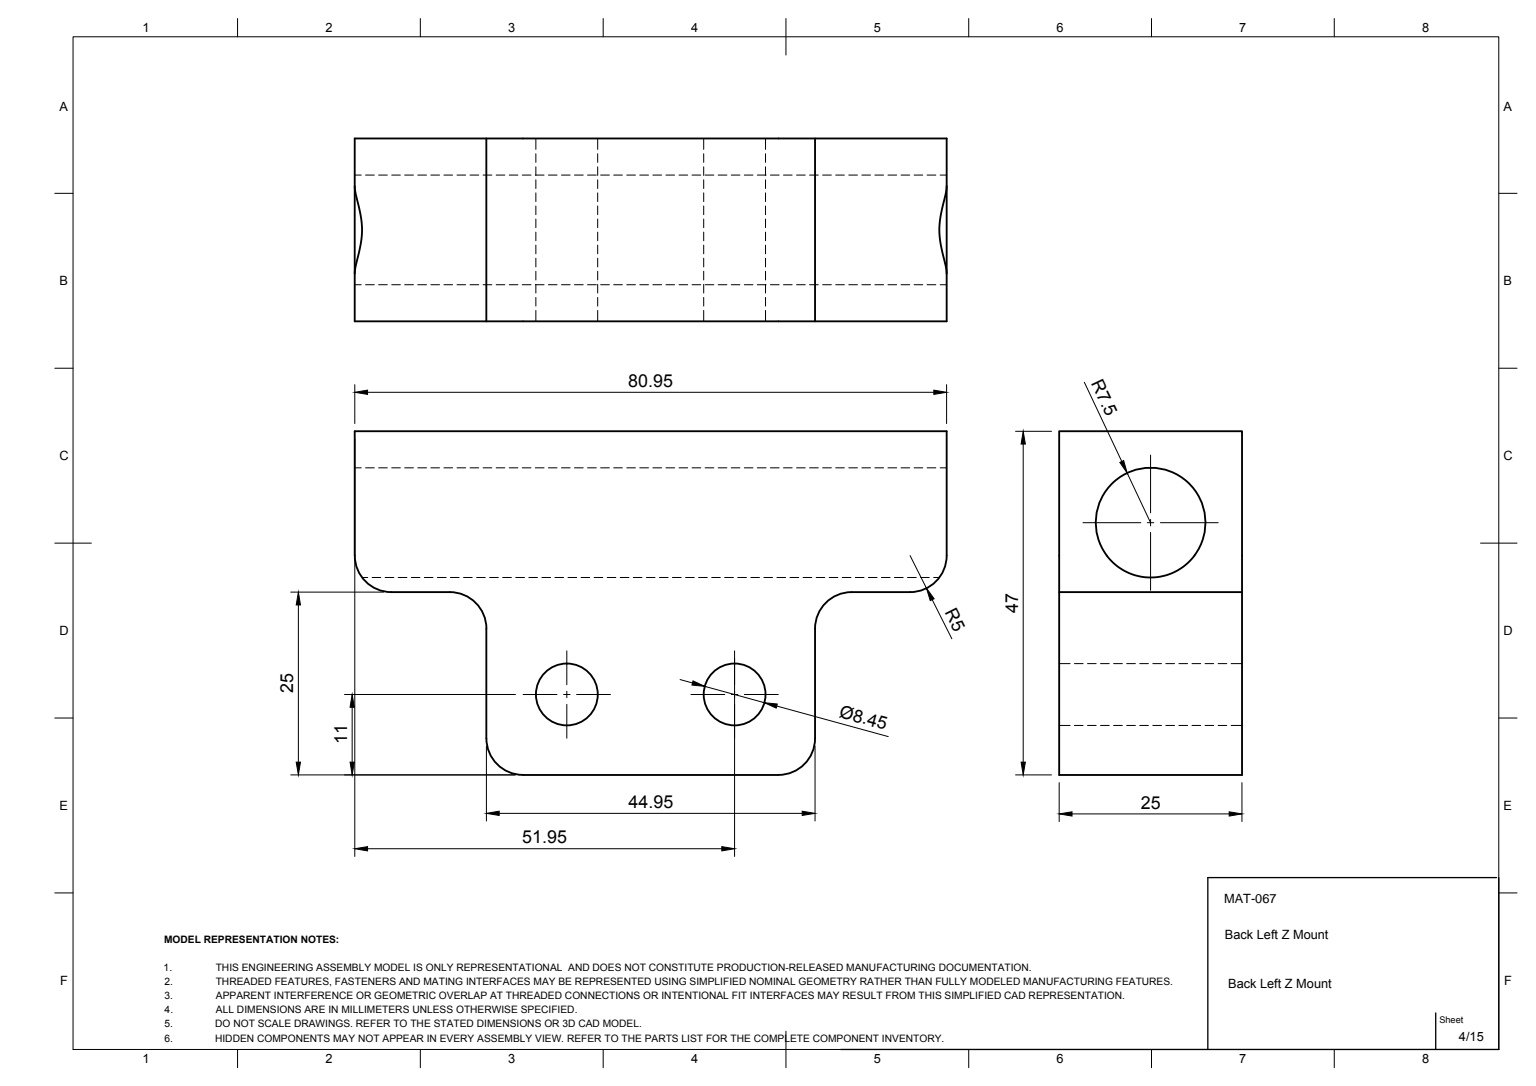
ISO-10303-21;
HEADER;
/* Generated by software containing ST-Developer
 * from STEP Tools, Inc. (www.steptools.com) 
 */

FILE_DESCRIPTION(
/* description */ ('CAx-IF Rec.Pracs.---Representation and Presentation of Product Manufa
cturing Information (PMI)---4.0---2014-10-13'),
/* implementation_level */ '2;1');

FILE_NAME(
/* name */ 'Back Left Z Mount.step',
/* time_stamp */ '2026-10-24T16:02:03-07:00',
/* author */ (''),
/* organization */ (''),
/* preprocessor_version */ 'ST-DEVELOPER v20.2',
/* originating_system */ 'Autodesk Translation Framework v15.17.0.0',
/* authorisation */ '');

FILE_SCHEMA (('AP242_MANAGED_MODEL_BASED_3D_ENGINEERING_MIM_LF { 1 0 10303 442 2 1 4 }'));
ENDSEC;

DATA;
#10=MECHANICAL_DESIGN_GEOMETRIC_PRESENTATION_REPRESENTATION('',(#350),#6348);
#328=SHAPE_REPRESENTATION_RELATIONSHIP('SRR','None',#6478,#339);
#339=ADVANCED_BREP_SHAPE_REPRESENTATION('',(#361),#6326);
#350=STYLED_ITEM('',(#6602),#361);
#361=MANIFOLD_SOLID_BREP('Body1',#3389);
#373=B_SPLINE_CURVE_WITH_KNOTS('',3,(#5376,#5377,#5378,#5379,#5380,#5381,
#5382,#5383,#5384,#5385,#5386,#5387,#5388,#5389,#5390,#5391,#5392,#5393),
 .UNSPECIFIED.,.F.,.F.,(4,2,2,2,2,2,2,2,4),(3.70111917994048,3.77979672158967,
4.08163951097076,4.2325609056613,4.38348230035184,4.53440369504239,4.68532508973293,
4.98716787911402,5.06584542076321),.UNSPECIFIED.);
#374=B_SPLINE_CURVE_WITH_KNOTS('',3,(#5394,#5395,#5396,#5397,#5398,#5399,
#5400,#5401,#5402,#5403,#5404,#5405,#5406,#5407,#5408,#5409,#5410,#5411),
 .UNSPECIFIED.,.F.,.F.,(4,2,2,2,2,2,2,2,4),(0.778797646372586,0.857475188021775,
1.15931797740286,1.31023937209341,1.46116076678395,1.61208216147449,1.76300355616504,
2.06484634554612,2.14352388719531),.UNSPECIFIED.);
#394=CYLINDRICAL_SURFACE('',#3588,0.004225);
#395=CYLINDRICAL_SURFACE('',#3589,0.004225);
#396=CYLINDRICAL_SURFACE('',#3591,0.0075);
#397=CYLINDRICAL_SURFACE('',#3596,0.005);
#398=CYLINDRICAL_SURFACE('',#3597,0.005);
#399=CYLINDRICAL_SURFACE('',#3598,0.005);
#400=CYLINDRICAL_SURFACE('',#3599,0.005);
#401=CYLINDRICAL_SURFACE('',#3600,0.005);
#402=CYLINDRICAL_SURFACE('',#3601,0.005);
#468=FACE_BOUND('',#892,.T.);
#469=FACE_BOUND('',#893,.T.);
#470=FACE_BOUND('',#895,.T.);
#471=FACE_BOUND('',#896,.T.);
#526=CIRCLE('',#3565,0.0075);
#527=CIRCLE('',#3566,0.0075);
#528=CIRCLE('',#3568,0.0075);
#529=CIRCLE('',#3569,0.0075);
#530=CIRCLE('',#3571,0.005);
#531=CIRCLE('',#3572,0.005);
#532=CIRCLE('',#3573,0.005);
#533=CIRCLE('',#3574,0.005);
#534=CIRCLE('',#3575,0.005);
#535=CIRCLE('',#3576,0.005);
#536=CIRCLE('',#3577,0.004225);
#537=CIRCLE('',#3578,0.004225);
#538=CIRCLE('',#3580,0.005);
#539=CIRCLE('',#3581,0.005);
#540=CIRCLE('',#3582,0.005);
#541=CIRCLE('',#3583,0.005);
#542=CIRCLE('',#3584,0.005);
#543=CIRCLE('',#3585,0.005);
#544=CIRCLE('',#3586,0.004225);
#545=CIRCLE('',#3587,0.004225);
#713=FACE_OUTER_BOUND('',#888,.T.);
#714=FACE_OUTER_BOUND('',#889,.T.);
#715=FACE_OUTER_BOUND('',#890,.T.);
#716=FACE_OUTER_BOUND('',#891,.T.);
#717=FACE_OUTER_BOUND('',#894,.T.);
#718=FACE_OUTER_BOUND('',#897,.T.);
#719=FACE_OUTER_BOUND('',#898,.T.);
#720=FACE_OUTER_BOUND('',#899,.T.);
#721=FACE_OUTER_BOUND('',#900,.T.);
#722=FACE_OUTER_BOUND('',#901,.T.);
#723=FACE_OUTER_BOUND('',#902,.T.);
#724=FACE_OUTER_BOUND('',#903,.T.);
#725=FACE_OUTER_BOUND('',#904,.T.);
#726=FACE_OUTER_BOUND('',#905,.T.);
#727=FACE_OUTER_BOUND('',#906,.T.);
#728=FACE_OUTER_BOUND('',#907,.T.);
#729=FACE_OUTER_BOUND('',#908,.T.);
#730=FACE_OUTER_BOUND('',#909,.T.);
#731=FACE_OUTER_BOUND('',#910,.T.);
#888=EDGE_LOOP('',(#2381,#2382,#2383,#2384));
#889=EDGE_LOOP('',(#2385,#2386,#2387,#2388,#2389,#2390,#2391));
#890=EDGE_LOOP('',(#2392,#2393,#2394,#2395,#2396,#2397,#2398));
#891=EDGE_LOOP('',(#2399,#2400,#2401,#2402,#2403,#2404,#2405,#2406,#2407,
#2408,#2409,#2410,#2411,#2412));
#892=EDGE_LOOP('',(#2413));
#893=EDGE_LOOP('',(#2414));
#894=EDGE_LOOP('',(#2415,#2416,#2417,#2418,#2419,#2420,#2421,#2422,#2423,
#2424,#2425,#2426,#2427,#2428));
#895=EDGE_LOOP('',(#2429));
#896=EDGE_LOOP('',(#2430));
#897=EDGE_LOOP('',(#2431,#2432,#2433,#2434));
#898=EDGE_LOOP('',(#2435,#2436,#2437,#2438));
#899=EDGE_LOOP('',(#2439,#2440,#2441,#2442));
#900=EDGE_LOOP('',(#2443,#2444,#2445,#2446,#2447,#2448,#2449,#2450));
#901=EDGE_LOOP('',(#2451,#2452,#2453,#2454));
#902=EDGE_LOOP('',(#2455,#2456,#2457,#2458));
#903=EDGE_LOOP('',(#2459,#2460,#2461,#2462));
#904=EDGE_LOOP('',(#2463,#2464,#2465,#2466));
#905=EDGE_LOOP('',(#2467,#2468,#2469,#2470));
#906=EDGE_LOOP('',(#2471,#2472,#2473,#2474,#2475,#2476));
#907=EDGE_LOOP('',(#2477,#2478,#2479,#2480));
#908=EDGE_LOOP('',(#2481,#2482,#2483,#2484,#2485,#2486));
#909=EDGE_LOOP('',(#2487,#2488,#2489,#2490));
#910=EDGE_LOOP('',(#2491,#2492,#2493,#2494));
#1113=LINE('',#5285,#1346);
#1114=LINE('',#5287,#1347);
#1115=LINE('',#5289,#1348);
#1116=LINE('',#5290,#1349);
#1117=LINE('',#5294,#1350);
#1118=LINE('',#5296,#1351);
#1119=LINE('',#5298,#1352);
#1120=LINE('',#5300,#1353);
#1121=LINE('',#5305,#1354);
#1122=LINE('',#5309,#1355);
#1123=LINE('',#5311,#1356);
#1124=LINE('',#5313,#1357);
#1125=LINE('',#5315,#1358);
#1126=LINE('',#5320,#1359);
#1127=LINE('',#5325,#1360);
#1128=LINE('',#5329,#1361);
#1129=LINE('',#5331,#1362);
#1130=LINE('',#5335,#1363);
#1131=LINE('',#5339,#1364);
#1132=LINE('',#5348,#1365);
#1133=LINE('',#5352,#1366);
#1134=LINE('',#5354,#1367);
#1135=LINE('',#5358,#1368);
#1136=LINE('',#5362,#1369);
#1137=LINE('',#5370,#1370);
#1138=LINE('',#5372,#1371);
#1139=LINE('',#5375,#1372);
#1140=LINE('',#5413,#1373);
#1141=LINE('',#5414,#1374);
#1142=LINE('',#5416,#1375);
#1143=LINE('',#5417,#1376);
#1144=LINE('',#5419,#1377);
#1145=LINE('',#5420,#1378);
#1146=LINE('',#5422,#1379);
#1147=LINE('',#5423,#1380);
#1346=VECTOR('',#4101,1.);
#1347=VECTOR('',#4102,1.);
#1348=VECTOR('',#4103,1.);
#1349=VECTOR('',#4104,1.);
#1350=VECTOR('',#4107,1.);
#1351=VECTOR('',#4108,1.);
#1352=VECTOR('',#4109,1.);
#1353=VECTOR('',#4110,1.);
#1354=VECTOR('',#4115,1.);
#1355=VECTOR('',#4118,1.);
#1356=VECTOR('',#4119,1.);
#1357=VECTOR('',#4120,1.);
#1358=VECTOR('',#4121,1.);
#1359=VECTOR('',#4126,1.);
#1360=VECTOR('',#4131,1.);
#1361=VECTOR('',#4134,1.);
#1362=VECTOR('',#4137,1.);
#1363=VECTOR('',#4140,1.);
#1364=VECTOR('',#4143,1.);
#1365=VECTOR('',#4152,1.);
#1366=VECTOR('',#4155,1.);
#1367=VECTOR('',#4158,1.);
#1368=VECTOR('',#4161,1.);
#1369=VECTOR('',#4164,1.);
#1370=VECTOR('',#4175,0.004225);
#1371=VECTOR('',#4178,0.004225);
#1372=VECTOR('',#4183,0.0075);
#1373=VECTOR('',#4186,1.);
#1374=VECTOR('',#4187,1.);
#1375=VECTOR('',#4190,1.);
#1376=VECTOR('',#4191,1.);
#1377=VECTOR('',#4194,1.);
#1378=VECTOR('',#4195,1.);
#1379=VECTOR('',#4198,1.);
#1380=VECTOR('',#4199,1.);
#1582=VERTEX_POINT('',#5283);
#1583=VERTEX_POINT('',#5284);
#1584=VERTEX_POINT('',#5286);
#1585=VERTEX_POINT('',#5288);
#1586=VERTEX_POINT('',#5292);
#1587=VERTEX_POINT('',#5293);
#1588=VERTEX_POINT('',#5295);
#1589=VERTEX_POINT('',#5297);
#1590=VERTEX_POINT('',#5299);
#1591=VERTEX_POINT('',#5301);
#1592=VERTEX_POINT('',#5303);
#1593=VERTEX_POINT('',#5307);
#1594=VERTEX_POINT('',#5308);
#1595=VERTEX_POINT('',#5310);
#1596=VERTEX_POINT('',#5312);
#1597=VERTEX_POINT('',#5314);
#1598=VERTEX_POINT('',#5316);
#1599=VERTEX_POINT('',#5318);
#1600=VERTEX_POINT('',#5322);
#1601=VERTEX_POINT('',#5324);
#1602=VERTEX_POINT('',#5326);
#1603=VERTEX_POINT('',#5328);
#1604=VERTEX_POINT('',#5332);
#1605=VERTEX_POINT('',#5334);
#1606=VERTEX_POINT('',#5336);
#1607=VERTEX_POINT('',#5338);
#1608=VERTEX_POINT('',#5341);
#1609=VERTEX_POINT('',#5343);
#1610=VERTEX_POINT('',#5346);
#1611=VERTEX_POINT('',#5347);
#1612=VERTEX_POINT('',#5349);
#1613=VERTEX_POINT('',#5351);
#1614=VERTEX_POINT('',#5355);
#1615=VERTEX_POINT('',#5357);
#1616=VERTEX_POINT('',#5359);
#1617=VERTEX_POINT('',#5361);
#1618=VERTEX_POINT('',#5365);
#1619=VERTEX_POINT('',#5367);
#1889=EDGE_CURVE('',#1582,#1583,#1113,.T.);
#1890=EDGE_CURVE('',#1584,#1582,#1114,.F.);
#1891=EDGE_CURVE('',#1584,#1585,#1115,.T.);
#1892=EDGE_CURVE('',#1583,#1585,#1116,.T.);
#1893=EDGE_CURVE('',#1586,#1587,#1117,.T.);
#1894=EDGE_CURVE('',#1587,#1588,#1118,.T.);
#1895=EDGE_CURVE('',#1589,#1588,#1119,.T.);
#1896=EDGE_CURVE('',#1590,#1589,#1120,.F.);
#1897=EDGE_CURVE('',#1591,#1590,#526,.T.);
#1898=EDGE_CURVE('',#1592,#1591,#527,.T.);
#1899=EDGE_CURVE('',#1586,#1592,#1121,.F.);
#1900=EDGE_CURVE('',#1593,#1594,#1122,.T.);
#1901=EDGE_CURVE('',#1595,#1594,#1123,.T.);
#1902=EDGE_CURVE('',#1596,#1595,#1124,.T.);
#1903=EDGE_CURVE('',#1597,#1596,#1125,.T.);
#1904=EDGE_CURVE('',#1597,#1598,#528,.T.);
#1905=EDGE_CURVE('',#1598,#1599,#529,.T.);
#1906=EDGE_CURVE('',#1593,#1599,#1126,.T.);
#1907=EDGE_CURVE('',#1600,#1584,#530,.T.);
#1908=EDGE_CURVE('',#1600,#1601,#1127,.T.);
#1909=EDGE_CURVE('',#1602,#1601,#531,.F.);
#1910=EDGE_CURVE('',#1603,#1602,#1128,.T.);
#1911=EDGE_CURVE('',#1596,#1603,#532,.T.);
#1912=EDGE_CURVE('',#1595,#1587,#1129,.T.);
#1913=EDGE_CURVE('',#1604,#1586,#533,.T.);
#1914=EDGE_CURVE('',#1604,#1605,#1130,.T.);
#1915=EDGE_CURVE('',#1606,#1605,#534,.F.);
#1916=EDGE_CURVE('',#1607,#1606,#1131,.T.);
#1917=EDGE_CURVE('',#1585,#1607,#535,.T.);
#1918=EDGE_CURVE('',#1608,#1608,#536,.T.);
#1919=EDGE_CURVE('',#1609,#1609,#537,.T.);
#1920=EDGE_CURVE('',#1610,#1611,#1132,.T.);
#1921=EDGE_CURVE('',#1612,#1611,#538,.T.);
#1922=EDGE_CURVE('',#1613,#1612,#1133,.T.);
#1923=EDGE_CURVE('',#1589,#1613,#539,.F.);
#1924=EDGE_CURVE('',#1594,#1588,#1134,.T.);
#1925=EDGE_CURVE('',#1614,#1593,#540,.F.);
#1926=EDGE_CURVE('',#1614,#1615,#1135,.T.);
#1927=EDGE_CURVE('',#1616,#1615,#541,.T.);
#1928=EDGE_CURVE('',#1617,#1616,#1136,.T.);
#1929=EDGE_CURVE('',#1582,#1617,#542,.F.);
#1930=EDGE_CURVE('',#1610,#1583,#543,.F.);
#1931=EDGE_CURVE('',#1618,#1618,#544,.T.);
#1932=EDGE_CURVE('',#1619,#1619,#545,.T.);
#1933=EDGE_CURVE('',#1608,#1618,#1137,.T.);
#1934=EDGE_CURVE('',#1609,#1619,#1138,.T.);
#1935=EDGE_CURVE('',#1591,#1598,#1139,.T.);
#1936=EDGE_CURVE('',#1599,#1597,#373,.T.);
#1937=EDGE_CURVE('',#1592,#1590,#374,.T.);
#1938=EDGE_CURVE('',#1611,#1606,#1140,.T.);
#1939=EDGE_CURVE('',#1607,#1610,#1141,.F.);
#1940=EDGE_CURVE('',#1605,#1612,#1142,.F.);
#1941=EDGE_CURVE('',#1613,#1604,#1143,.T.);
#1942=EDGE_CURVE('',#1617,#1600,#1144,.T.);
#1943=EDGE_CURVE('',#1601,#1616,#1145,.F.);
#1944=EDGE_CURVE('',#1615,#1602,#1146,.T.);
#1945=EDGE_CURVE('',#1603,#1614,#1147,.F.);
#2381=ORIENTED_EDGE('',*,*,#1889,.F.);
#2382=ORIENTED_EDGE('',*,*,#1890,.F.);
#2383=ORIENTED_EDGE('',*,*,#1891,.T.);
#2384=ORIENTED_EDGE('',*,*,#1892,.F.);
#2385=ORIENTED_EDGE('',*,*,#1893,.T.);
#2386=ORIENTED_EDGE('',*,*,#1894,.T.);
#2387=ORIENTED_EDGE('',*,*,#1895,.F.);
#2388=ORIENTED_EDGE('',*,*,#1896,.F.);
#2389=ORIENTED_EDGE('',*,*,#1897,.F.);
#2390=ORIENTED_EDGE('',*,*,#1898,.F.);
#2391=ORIENTED_EDGE('',*,*,#1899,.F.);
#2392=ORIENTED_EDGE('',*,*,#1900,.T.);
#2393=ORIENTED_EDGE('',*,*,#1901,.F.);
#2394=ORIENTED_EDGE('',*,*,#1902,.F.);
#2395=ORIENTED_EDGE('',*,*,#1903,.F.);
#2396=ORIENTED_EDGE('',*,*,#1904,.T.);
#2397=ORIENTED_EDGE('',*,*,#1905,.T.);
#2398=ORIENTED_EDGE('',*,*,#1906,.F.);
#2399=ORIENTED_EDGE('',*,*,#1891,.F.);
#2400=ORIENTED_EDGE('',*,*,#1907,.F.);
#2401=ORIENTED_EDGE('',*,*,#1908,.T.);
#2402=ORIENTED_EDGE('',*,*,#1909,.F.);
#2403=ORIENTED_EDGE('',*,*,#1910,.F.);
#2404=ORIENTED_EDGE('',*,*,#1911,.F.);
#2405=ORIENTED_EDGE('',*,*,#1902,.T.);
#2406=ORIENTED_EDGE('',*,*,#1912,.T.);
#2407=ORIENTED_EDGE('',*,*,#1893,.F.);
#2408=ORIENTED_EDGE('',*,*,#1913,.F.);
#2409=ORIENTED_EDGE('',*,*,#1914,.T.);
#2410=ORIENTED_EDGE('',*,*,#1915,.F.);
#2411=ORIENTED_EDGE('',*,*,#1916,.F.);
#2412=ORIENTED_EDGE('',*,*,#1917,.F.);
#2413=ORIENTED_EDGE('',*,*,#1918,.T.);
#2414=ORIENTED_EDGE('',*,*,#1919,.T.);
#2415=ORIENTED_EDGE('',*,*,#1920,.T.);
#2416=ORIENTED_EDGE('',*,*,#1921,.F.);
#2417=ORIENTED_EDGE('',*,*,#1922,.F.);
#2418=ORIENTED_EDGE('',*,*,#1923,.F.);
#2419=ORIENTED_EDGE('',*,*,#1895,.T.);
#2420=ORIENTED_EDGE('',*,*,#1924,.F.);
#2421=ORIENTED_EDGE('',*,*,#1900,.F.);
#2422=ORIENTED_EDGE('',*,*,#1925,.F.);
#2423=ORIENTED_EDGE('',*,*,#1926,.T.);
#2424=ORIENTED_EDGE('',*,*,#1927,.F.);
#2425=ORIENTED_EDGE('',*,*,#1928,.F.);
#2426=ORIENTED_EDGE('',*,*,#1929,.F.);
#2427=ORIENTED_EDGE('',*,*,#1889,.T.);
#2428=ORIENTED_EDGE('',*,*,#1930,.F.);
#2429=ORIENTED_EDGE('',*,*,#1931,.F.);
#2430=ORIENTED_EDGE('',*,*,#1932,.F.);
#2431=ORIENTED_EDGE('',*,*,#1918,.F.);
#2432=ORIENTED_EDGE('',*,*,#1933,.T.);
#2433=ORIENTED_EDGE('',*,*,#1931,.T.);
#2434=ORIENTED_EDGE('',*,*,#1933,.F.);
#2435=ORIENTED_EDGE('',*,*,#1919,.F.);
#2436=ORIENTED_EDGE('',*,*,#1934,.T.);
#2437=ORIENTED_EDGE('',*,*,#1932,.T.);
#2438=ORIENTED_EDGE('',*,*,#1934,.F.);
#2439=ORIENTED_EDGE('',*,*,#1924,.T.);
#2440=ORIENTED_EDGE('',*,*,#1894,.F.);
#2441=ORIENTED_EDGE('',*,*,#1912,.F.);
#2442=ORIENTED_EDGE('',*,*,#1901,.T.);
#2443=ORIENTED_EDGE('',*,*,#1898,.T.);
#2444=ORIENTED_EDGE('',*,*,#1935,.T.);
#2445=ORIENTED_EDGE('',*,*,#1904,.F.);
#2446=ORIENTED_EDGE('',*,*,#1936,.F.);
#2447=ORIENTED_EDGE('',*,*,#1905,.F.);
#2448=ORIENTED_EDGE('',*,*,#1935,.F.);
#2449=ORIENTED_EDGE('',*,*,#1897,.T.);
#2450=ORIENTED_EDGE('',*,*,#1937,.F.);
#2451=ORIENTED_EDGE('',*,*,#1916,.T.);
#2452=ORIENTED_EDGE('',*,*,#1938,.F.);
#2453=ORIENTED_EDGE('',*,*,#1920,.F.);
#2454=ORIENTED_EDGE('',*,*,#1939,.F.);
#2455=ORIENTED_EDGE('',*,*,#1922,.T.);
#2456=ORIENTED_EDGE('',*,*,#1940,.F.);
#2457=ORIENTED_EDGE('',*,*,#1914,.F.);
#2458=ORIENTED_EDGE('',*,*,#1941,.F.);
#2459=ORIENTED_EDGE('',*,*,#1908,.F.);
#2460=ORIENTED_EDGE('',*,*,#1942,.F.);
#2461=ORIENTED_EDGE('',*,*,#1928,.T.);
#2462=ORIENTED_EDGE('',*,*,#1943,.F.);
#2463=ORIENTED_EDGE('',*,*,#1910,.T.);
#2464=ORIENTED_EDGE('',*,*,#1944,.F.);
#2465=ORIENTED_EDGE('',*,*,#1926,.F.);
#2466=ORIENTED_EDGE('',*,*,#1945,.F.);
#2467=ORIENTED_EDGE('',*,*,#1930,.T.);
#2468=ORIENTED_EDGE('',*,*,#1892,.T.);
#2469=ORIENTED_EDGE('',*,*,#1917,.T.);
#2470=ORIENTED_EDGE('',*,*,#1939,.T.);
#2471=ORIENTED_EDGE('',*,*,#1937,.T.);
#2472=ORIENTED_EDGE('',*,*,#1896,.T.);
#2473=ORIENTED_EDGE('',*,*,#1923,.T.);
#2474=ORIENTED_EDGE('',*,*,#1941,.T.);
#2475=ORIENTED_EDGE('',*,*,#1913,.T.);
#2476=ORIENTED_EDGE('',*,*,#1899,.T.);
#2477=ORIENTED_EDGE('',*,*,#1921,.T.);
#2478=ORIENTED_EDGE('',*,*,#1938,.T.);
#2479=ORIENTED_EDGE('',*,*,#1915,.T.);
#2480=ORIENTED_EDGE('',*,*,#1940,.T.);
#2481=ORIENTED_EDGE('',*,*,#1925,.T.);
#2482=ORIENTED_EDGE('',*,*,#1906,.T.);
#2483=ORIENTED_EDGE('',*,*,#1936,.T.);
#2484=ORIENTED_EDGE('',*,*,#1903,.T.);
#2485=ORIENTED_EDGE('',*,*,#1911,.T.);
#2486=ORIENTED_EDGE('',*,*,#1945,.T.);
#2487=ORIENTED_EDGE('',*,*,#1927,.T.);
#2488=ORIENTED_EDGE('',*,*,#1944,.T.);
#2489=ORIENTED_EDGE('',*,*,#1909,.T.);
#2490=ORIENTED_EDGE('',*,*,#1943,.T.);
#2491=ORIENTED_EDGE('',*,*,#1929,.T.);
#2492=ORIENTED_EDGE('',*,*,#1942,.T.);
#2493=ORIENTED_EDGE('',*,*,#1907,.T.);
#2494=ORIENTED_EDGE('',*,*,#1890,.T.);
#3147=PLANE('',#3563);
#3148=PLANE('',#3564);
#3149=PLANE('',#3567);
#3150=PLANE('',#3570);
#3151=PLANE('',#3579);
#3152=PLANE('',#3590);
#3153=PLANE('',#3592);
#3154=PLANE('',#3593);
#3155=PLANE('',#3594);
#3156=PLANE('',#3595);
#3236=ADVANCED_FACE('',(#713),#3147,.F.);
#3237=ADVANCED_FACE('',(#714),#3148,.F.);
#3238=ADVANCED_FACE('',(#715),#3149,.T.);
#3239=ADVANCED_FACE('',(#716,#468,#469),#3150,.T.);
#3240=ADVANCED_FACE('',(#717,#470,#471),#3151,.F.);
#3241=ADVANCED_FACE('',(#718),#394,.F.);
#3242=ADVANCED_FACE('',(#719),#395,.F.);
#3243=ADVANCED_FACE('',(#720),#3152,.T.);
#3244=ADVANCED_FACE('',(#721),#396,.F.);
#3245=ADVANCED_FACE('',(#722),#3153,.T.);
#3246=ADVANCED_FACE('',(#723),#3154,.F.);
#3247=ADVANCED_FACE('',(#724),#3155,.F.);
#3248=ADVANCED_FACE('',(#725),#3156,.T.);
#3249=ADVANCED_FACE('',(#726),#397,.T.);
#3250=ADVANCED_FACE('',(#727),#398,.T.);
#3251=ADVANCED_FACE('',(#728),#399,.F.);
#3252=ADVANCED_FACE('',(#729),#400,.T.);
#3253=ADVANCED_FACE('',(#730),#401,.F.);
#3254=ADVANCED_FACE('',(#731),#402,.T.);
#3389=CLOSED_SHELL('',(#3236,#3237,#3238,#3239,#3240,#3241,#3242,#3243,
#3244,#3245,#3246,#3247,#3248,#3249,#3250,#3251,#3252,#3253,#3254));
#3562=AXIS2_PLACEMENT_3D('',#5281,#4097,#4098);
#3563=AXIS2_PLACEMENT_3D('',#5282,#4099,#4100);
#3564=AXIS2_PLACEMENT_3D('',#5291,#4105,#4106);
#3565=AXIS2_PLACEMENT_3D('',#5302,#4111,#4112);
#3566=AXIS2_PLACEMENT_3D('',#5304,#4113,#4114);
#3567=AXIS2_PLACEMENT_3D('',#5306,#4116,#4117);
#3568=AXIS2_PLACEMENT_3D('',#5317,#4122,#4123);
#3569=AXIS2_PLACEMENT_3D('',#5319,#4124,#4125);
#3570=AXIS2_PLACEMENT_3D('',#5321,#4127,#4128);
#3571=AXIS2_PLACEMENT_3D('',#5323,#4129,#4130);
#3572=AXIS2_PLACEMENT_3D('',#5327,#4132,#4133);
#3573=AXIS2_PLACEMENT_3D('',#5330,#4135,#4136);
#3574=AXIS2_PLACEMENT_3D('',#5333,#4138,#4139);
#3575=AXIS2_PLACEMENT_3D('',#5337,#4141,#4142);
#3576=AXIS2_PLACEMENT_3D('',#5340,#4144,#4145);
#3577=AXIS2_PLACEMENT_3D('',#5342,#4146,#4147);
#3578=AXIS2_PLACEMENT_3D('',#5344,#4148,#4149);
#3579=AXIS2_PLACEMENT_3D('',#5345,#4150,#4151);
#3580=AXIS2_PLACEMENT_3D('',#5350,#4153,#4154);
#3581=AXIS2_PLACEMENT_3D('',#5353,#4156,#4157);
#3582=AXIS2_PLACEMENT_3D('',#5356,#4159,#4160);
#3583=AXIS2_PLACEMENT_3D('',#5360,#4162,#4163);
#3584=AXIS2_PLACEMENT_3D('',#5363,#4165,#4166);
#3585=AXIS2_PLACEMENT_3D('',#5364,#4167,#4168);
#3586=AXIS2_PLACEMENT_3D('',#5366,#4169,#4170);
#3587=AXIS2_PLACEMENT_3D('',#5368,#4171,#4172);
#3588=AXIS2_PLACEMENT_3D('',#5369,#4173,#4174);
#3589=AXIS2_PLACEMENT_3D('',#5371,#4176,#4177);
#3590=AXIS2_PLACEMENT_3D('',#5373,#4179,#4180);
#3591=AXIS2_PLACEMENT_3D('',#5374,#4181,#4182);
#3592=AXIS2_PLACEMENT_3D('',#5412,#4184,#4185);
#3593=AXIS2_PLACEMENT_3D('',#5415,#4188,#4189);
#3594=AXIS2_PLACEMENT_3D('',#5418,#4192,#4193);
#3595=AXIS2_PLACEMENT_3D('',#5421,#4196,#4197);
#3596=AXIS2_PLACEMENT_3D('',#5424,#4200,#4201);
#3597=AXIS2_PLACEMENT_3D('',#5425,#4202,#4203);
#3598=AXIS2_PLACEMENT_3D('',#5426,#4204,#4205);
#3599=AXIS2_PLACEMENT_3D('',#5427,#4206,#4207);
#3600=AXIS2_PLACEMENT_3D('',#5428,#4208,#4209);
#3601=AXIS2_PLACEMENT_3D('',#5429,#4210,#4211);
#4097=DIRECTION('axis',(0.,0.,1.));
#4098=DIRECTION('refdir',(1.,0.,0.));
#4099=DIRECTION('center_axis',(1.,0.,0.));
#4100=DIRECTION('ref_axis',(0.,0.,-1.));
#4101=DIRECTION('',(0.,8.57182693503055E-17,-1.));
#4102=DIRECTION('',(0.,1.,8.57182693503055E-17));
#4103=DIRECTION('',(0.,8.57182693503055E-17,-1.));
#4104=DIRECTION('',(0.,1.,8.57182693503055E-17));
#4105=DIRECTION('center_axis',(0.,-8.57182693503055E-17,1.));
#4106=DIRECTION('ref_axis',(0.,1.,8.57182693503055E-17));
#4107=DIRECTION('',(1.,0.,0.));
#4108=DIRECTION('',(0.,-1.,-8.57182693503055E-17));
#4109=DIRECTION('',(1.,0.,0.));
#4110=DIRECTION('',(0.,1.,8.57182693503055E-17));
#4111=DIRECTION('center_axis',(0.,8.57182693503055E-17,-1.));
#4112=DIRECTION('ref_axis',(0.,1.,8.57182693503055E-17));
#4113=DIRECTION('center_axis',(0.,8.57182693503055E-17,-1.));
#4114=DIRECTION('ref_axis',(0.,1.,8.57182693503055E-17));
#4115=DIRECTION('',(0.,1.,8.57182693503055E-17));
#4116=DIRECTION('center_axis',(0.,-8.57182693503055E-17,1.));
#4117=DIRECTION('ref_axis',(0.,1.,8.57182693503055E-17));
#4118=DIRECTION('',(1.,0.,0.));
#4119=DIRECTION('',(0.,-1.,-8.57182693503055E-17));
#4120=DIRECTION('',(1.,0.,0.));
#4121=DIRECTION('',(0.,1.,8.57182693503055E-17));
#4122=DIRECTION('center_axis',(0.,8.57182693503055E-17,-1.));
#4123=DIRECTION('ref_axis',(0.,1.,8.57182693503055E-17));
#4124=DIRECTION('center_axis',(0.,8.57182693503055E-17,-1.));
#4125=DIRECTION('ref_axis',(0.,1.,8.57182693503055E-17));
#4126=DIRECTION('',(0.,1.,8.57182693503055E-17));
#4127=DIRECTION('center_axis',(0.,1.,8.57182693503055E-17));
#4128=DIRECTION('ref_axis',(1.,0.,0.));
#4129=DIRECTION('center_axis',(0.,-1.,-8.57182693503055E-17));
#4130=DIRECTION('ref_axis',(0.,8.57182693503055E-17,-1.));
#4131=DIRECTION('',(1.,0.,0.));
#4132=DIRECTION('center_axis',(0.,-1.,-8.57182693503055E-17));
#4133=DIRECTION('ref_axis',(0.,8.57182693503055E-17,-1.));
#4134=DIRECTION('',(0.,8.57182693503055E-17,-1.));
#4135=DIRECTION('center_axis',(0.,-1.,-8.57182693503055E-17));
#4136=DIRECTION('ref_axis',(0.,8.57182693503055E-17,-1.));
#4137=DIRECTION('',(0.,8.57182693503055E-17,-1.));
#4138=DIRECTION('center_axis',(0.,-1.,-8.57182693503055E-17));
#4139=DIRECTION('ref_axis',(0.,8.57182693503055E-17,-1.));
#4140=DIRECTION('',(0.,-8.57182693503055E-17,1.));
#4141=DIRECTION('center_axis',(0.,-1.,-8.57182693503055E-17));
#4142=DIRECTION('ref_axis',(0.,8.57182693503055E-17,-1.));
#4143=DIRECTION('',(1.,0.,0.));
#4144=DIRECTION('center_axis',(0.,-1.,-8.57182693503055E-17));
#4145=DIRECTION('ref_axis',(0.,8.57182693503055E-17,-1.));
#4146=DIRECTION('center_axis',(0.,-1.,-8.57182693503055E-17));
#4147=DIRECTION('ref_axis',(0.,8.57182693503055E-17,-1.));
#4148=DIRECTION('center_axis',(0.,-1.,-8.57182693503055E-17));
#4149=DIRECTION('ref_axis',(0.,8.57182693503055E-17,-1.));
#4150=DIRECTION('center_axis',(0.,1.,8.57182693503055E-17));
#4151=DIRECTION('ref_axis',(1.,0.,0.));
#4152=DIRECTION('',(1.,0.,0.));
#4153=DIRECTION('center_axis',(0.,-1.,-8.57182693503055E-17));
#4154=DIRECTION('ref_axis',(0.,8.57182693503055E-17,-1.));
#4155=DIRECTION('',(0.,-8.57182693503055E-17,1.));
#4156=DIRECTION('center_axis',(0.,-1.,-8.57182693503055E-17));
#4157=DIRECTION('ref_axis',(0.,8.57182693503055E-17,-1.));
#4158=DIRECTION('',(0.,8.57182693503055E-17,-1.));
#4159=DIRECTION('center_axis',(0.,-1.,-8.57182693503055E-17));
#4160=DIRECTION('ref_axis',(0.,8.57182693503055E-17,-1.));
#4161=DIRECTION('',(0.,8.57182693503055E-17,-1.));
#4162=DIRECTION('center_axis',(0.,-1.,-8.57182693503055E-17));
#4163=DIRECTION('ref_axis',(0.,8.57182693503055E-17,-1.));
#4164=DIRECTION('',(1.,0.,0.));
#4165=DIRECTION('center_axis',(0.,-1.,-8.57182693503055E-17));
#4166=DIRECTION('ref_axis',(0.,8.57182693503055E-17,-1.));
#4167=DIRECTION('center_axis',(0.,-1.,-8.57182693503055E-17));
#4168=DIRECTION('ref_axis',(0.,8.57182693503055E-17,-1.));
#4169=DIRECTION('center_axis',(0.,-1.,-8.57182693503055E-17));
#4170=DIRECTION('ref_axis',(0.,8.57182693503055E-17,-1.));
#4171=DIRECTION('center_axis',(0.,-1.,-8.57182693503055E-17));
#4172=DIRECTION('ref_axis',(0.,8.57182693503055E-17,-1.));
#4173=DIRECTION('center_axis',(0.,-1.,-8.57182693503055E-17));
#4174=DIRECTION('ref_axis',(0.,-8.57182693503055E-17,1.));
#4175=DIRECTION('',(0.,-1.,-8.57182693503055E-17));
#4176=DIRECTION('center_axis',(0.,-1.,-8.57182693503055E-17));
#4177=DIRECTION('ref_axis',(0.,-8.57182693503055E-17,1.));
#4178=DIRECTION('',(0.,-1.,-8.57182693503055E-17));
#4179=DIRECTION('center_axis',(1.,0.,0.));
#4180=DIRECTION('ref_axis',(0.,0.,-1.));
#4181=DIRECTION('center_axis',(0.,-8.57182693503055E-17,1.));
#4182=DIRECTION('ref_axis',(0.,1.,8.57182693503055E-17));
#4183=DIRECTION('',(0.,-8.57182693503055E-17,1.));
#4184=DIRECTION('center_axis',(0.,8.57182693503055E-17,-1.));
#4185=DIRECTION('ref_axis',(0.,-1.,-8.57182693503055E-17));
#4186=DIRECTION('',(0.,1.,8.57182693503055E-17));
#4187=DIRECTION('',(0.,1.,8.57182693503055E-17));
#4188=DIRECTION('center_axis',(1.,0.,0.));
#4189=DIRECTION('ref_axis',(0.,0.,-1.));
#4190=DIRECTION('',(0.,1.,8.57182693503055E-17));
#4191=DIRECTION('',(0.,1.,8.57182693503055E-17));
#4192=DIRECTION('center_axis',(0.,8.57182693503055E-17,-1.));
#4193=DIRECTION('ref_axis',(0.,-1.,-8.57182693503055E-17));
#4194=DIRECTION('',(0.,1.,8.57182693503055E-17));
#4195=DIRECTION('',(0.,1.,8.57182693503055E-17));
#4196=DIRECTION('center_axis',(-1.,0.,0.));
#4197=DIRECTION('ref_axis',(0.,0.,1.));
#4198=DIRECTION('',(0.,1.,8.57182693503055E-17));
#4199=DIRECTION('',(0.,1.,8.57182693503055E-17));
#4200=DIRECTION('center_axis',(0.,-1.,-8.57182693503055E-17));
#4201=DIRECTION('ref_axis',(0.,-8.57182693503055E-17,1.));
#4202=DIRECTION('center_axis',(0.,1.,8.57182693503055E-17));
#4203=DIRECTION('ref_axis',(0.,8.57182693503055E-17,-1.));
#4204=DIRECTION('center_axis',(0.,1.,8.57182693503055E-17));
#4205=DIRECTION('ref_axis',(0.,8.57182693503055E-17,-1.));
#4206=DIRECTION('center_axis',(0.,1.,8.57182693503055E-17));
#4207=DIRECTION('ref_axis',(0.,8.57182693503055E-17,-1.));
#4208=DIRECTION('center_axis',(0.,1.,8.57182693503055E-17));
#4209=DIRECTION('ref_axis',(0.,8.57182693503055E-17,-1.));
#4210=DIRECTION('center_axis',(0.,1.,8.57182693503055E-17));
#4211=DIRECTION('ref_axis',(0.,8.57182693503055E-17,-1.));
#5281=CARTESIAN_POINT('',(0.,0.,0.));
#5282=CARTESIAN_POINT('Origin',(-0.06855,0.1092,0.02565));
#5283=CARTESIAN_POINT('',(-0.06855,0.0842,0.043125));
#5284=CARTESIAN_POINT('',(-0.06855,0.0842,0.008175));
#5285=CARTESIAN_POINT('',(-0.06855,0.0842,0.02565));
#5286=CARTESIAN_POINT('',(-0.06855,0.1092,0.043125));
#5287=CARTESIAN_POINT('',(-0.06855,0.1092,0.043125));
#5288=CARTESIAN_POINT('',(-0.06855,0.1092,0.008175));
#5289=CARTESIAN_POINT('',(-0.06855,0.1092,0.02565));
#5290=CARTESIAN_POINT('',(-0.06855,0.1092,0.008175));
#5291=CARTESIAN_POINT('Origin',(-0.05755,0.1092,-0.014825));
#5292=CARTESIAN_POINT('',(-0.03855,0.1092,-0.014825));
#5293=CARTESIAN_POINT('',(-0.02155,0.1092,-0.014825));
#5294=CARTESIAN_POINT('',(-0.05755,0.1092,-0.014825));
#5295=CARTESIAN_POINT('',(-0.02155,0.0842,-0.014825));
#5296=CARTESIAN_POINT('',(-0.02155,0.1092,-0.014825));
#5297=CARTESIAN_POINT('',(-0.03855,0.0842,-0.014825));
#5298=CARTESIAN_POINT('',(-0.05755,0.0842,-0.014825));
#5299=CARTESIAN_POINT('',(-0.03855,0.0907,-0.014825));
#5300=CARTESIAN_POINT('',(-0.03855,0.1092,-0.014825));
#5301=CARTESIAN_POINT('',(-0.03405,0.0892,-0.014825));
#5302=CARTESIAN_POINT('Origin',(-0.03405,0.0967,-0.014825));
#5303=CARTESIAN_POINT('',(-0.03855,0.1027,-0.014825));
#5304=CARTESIAN_POINT('Origin',(-0.03405,0.0967,-0.014825));
#5305=CARTESIAN_POINT('',(-0.03855,0.1092,-0.014825));
#5306=CARTESIAN_POINT('Origin',(-0.05755,0.1092,0.066125));
#5307=CARTESIAN_POINT('',(-0.03855,0.0842,0.066125));
#5308=CARTESIAN_POINT('',(-0.02155,0.0842,0.066125));
#5309=CARTESIAN_POINT('',(-0.05755,0.0842,0.066125));
#5310=CARTESIAN_POINT('',(-0.02155,0.1092,0.066125));
#5311=CARTESIAN_POINT('',(-0.02155,0.1092,0.066125));
#5312=CARTESIAN_POINT('',(-0.03855,0.1092,0.066125));
#5313=CARTESIAN_POINT('',(-0.05755,0.1092,0.066125));
#5314=CARTESIAN_POINT('',(-0.03855,0.1027,0.066125));
#5315=CARTESIAN_POINT('',(-0.03855,0.1092,0.066125));
#5316=CARTESIAN_POINT('',(-0.03405,0.0892,0.066125));
#5317=CARTESIAN_POINT('Origin',(-0.03405,0.0967,0.066125));
#5318=CARTESIAN_POINT('',(-0.03855,0.0907,0.066125));
#5319=CARTESIAN_POINT('Origin',(-0.03405,0.0967,0.066125));
#5320=CARTESIAN_POINT('',(-0.03855,0.1092,0.066125));
#5321=CARTESIAN_POINT('Origin',(-0.05755,0.1092,0.02565));
#5322=CARTESIAN_POINT('',(-0.06355,0.1092,0.048125));
#5323=CARTESIAN_POINT('Origin',(-0.06355,0.1092,0.043125));
#5324=CARTESIAN_POINT('',(-0.04855,0.1092,0.048125));
#5325=CARTESIAN_POINT('',(-0.05605,0.1092,0.048125));
#5326=CARTESIAN_POINT('',(-0.04355,0.1092,0.053125));
#5327=CARTESIAN_POINT('Origin',(-0.04855,0.1092,0.053125));
#5328=CARTESIAN_POINT('',(-0.04355,0.1092,0.061125));
#5329=CARTESIAN_POINT('',(-0.04355,0.1092,0.057125));
#5330=CARTESIAN_POINT('Origin',(-0.03855,0.1092,0.061125));
#5331=CARTESIAN_POINT('',(-0.02155,0.1092,0.02565));
#5332=CARTESIAN_POINT('',(-0.04355,0.1092,-0.009825));
#5333=CARTESIAN_POINT('Origin',(-0.03855,0.1092,-0.009825));
#5334=CARTESIAN_POINT('',(-0.04355,0.1092,-0.001825));
#5335=CARTESIAN_POINT('',(-0.04355,0.1092,-0.005825));
#5336=CARTESIAN_POINT('',(-0.04855,0.1092,0.003175));
#5337=CARTESIAN_POINT('Origin',(-0.04855,0.1092,-0.001825));
#5338=CARTESIAN_POINT('',(-0.06355,0.1092,0.003175));
#5339=CARTESIAN_POINT('',(-0.05605,0.1092,0.003175));
#5340=CARTESIAN_POINT('Origin',(-0.06355,0.1092,0.008175));
#5341=CARTESIAN_POINT('',(-0.05755,0.1092,0.0329));
#5342=CARTESIAN_POINT('Origin',(-0.05755,0.1092,0.037125));
#5343=CARTESIAN_POINT('',(-0.05755,0.1092,0.00995));
#5344=CARTESIAN_POINT('Origin',(-0.05755,0.1092,0.014175));
#5345=CARTESIAN_POINT('Origin',(-0.05755,0.0842,0.02565));
#5346=CARTESIAN_POINT('',(-0.06355,0.0842,0.003175));
#5347=CARTESIAN_POINT('',(-0.04855,0.0842,0.003175));
#5348=CARTESIAN_POINT('',(-0.05605,0.0842,0.003175));
#5349=CARTESIAN_POINT('',(-0.04355,0.0842,-0.001825));
#5350=CARTESIAN_POINT('Origin',(-0.04855,0.0842,-0.001825));
#5351=CARTESIAN_POINT('',(-0.04355,0.0842,-0.009825));
#5352=CARTESIAN_POINT('',(-0.04355,0.0842,-0.005825));
#5353=CARTESIAN_POINT('Origin',(-0.03855,0.0842,-0.009825));
#5354=CARTESIAN_POINT('',(-0.02155,0.0842,0.02565));
#5355=CARTESIAN_POINT('',(-0.04355,0.0842,0.061125));
#5356=CARTESIAN_POINT('Origin',(-0.03855,0.0842,0.061125));
#5357=CARTESIAN_POINT('',(-0.04355,0.0842,0.053125));
#5358=CARTESIAN_POINT('',(-0.04355,0.0842,0.057125));
#5359=CARTESIAN_POINT('',(-0.04855,0.0842,0.048125));
#5360=CARTESIAN_POINT('Origin',(-0.04855,0.0842,0.053125));
#5361=CARTESIAN_POINT('',(-0.06355,0.0842,0.048125));
#5362=CARTESIAN_POINT('',(-0.05605,0.0842,0.048125));
#5363=CARTESIAN_POINT('Origin',(-0.06355,0.0842,0.043125));
#5364=CARTESIAN_POINT('Origin',(-0.06355,0.0842,0.008175));
#5365=CARTESIAN_POINT('',(-0.05755,0.0842,0.0329));
#5366=CARTESIAN_POINT('Origin',(-0.05755,0.0842,0.037125));
#5367=CARTESIAN_POINT('',(-0.05755,0.0842,0.00995));
#5368=CARTESIAN_POINT('Origin',(-0.05755,0.0842,0.014175));
#5369=CARTESIAN_POINT('Origin',(-0.05755,0.1092,0.037125));
#5370=CARTESIAN_POINT('',(-0.05755,0.1092,0.0329));
#5371=CARTESIAN_POINT('Origin',(-0.05755,0.1092,0.014175));
#5372=CARTESIAN_POINT('',(-0.05755,0.1092,0.00995));
#5373=CARTESIAN_POINT('Origin',(-0.02155,0.1092,0.02565));
#5374=CARTESIAN_POINT('Origin',(-0.03405,0.0967,-0.023875));
#5375=CARTESIAN_POINT('',(-0.03405,0.0892,-0.023875));
#5376=CARTESIAN_POINT('Ctrl Pts',(-0.03855,0.0907,0.066125));
#5377=CARTESIAN_POINT('Ctrl Pts',(-0.0387729524989471,0.0908672143742104,
0.066125));
#5378=CARTESIAN_POINT('Ctrl Pts',(-0.0389827504953742,0.0910443676288105,
0.0661099450879691));
#5379=CARTESIAN_POINT('Ctrl Pts',(-0.0399051826894431,0.0919072239369945,
0.0659940175331532));
#5380=CARTESIAN_POINT('Ctrl Pts',(-0.0405168708018142,0.0927639295079321,
0.0657455865368071));
#5381=CARTESIAN_POINT('Ctrl Pts',(-0.0411335425015076,0.0941822279651364,
0.0654121811456859));
#5382=CARTESIAN_POINT('Ctrl Pts',(-0.0412904479475092,0.0946775248634452,
0.0653090151899698));
#5383=CARTESIAN_POINT('Ctrl Pts',(-0.0414987473161672,0.0956847881043564,
0.065164916792468));
#5384=CARTESIAN_POINT('Ctrl Pts',(-0.04155,0.0961969286843649,0.065125));
#5385=CARTESIAN_POINT('Ctrl Pts',(-0.04155,0.0972030713156352,0.065125));
#5386=CARTESIAN_POINT('Ctrl Pts',(-0.0414987473161672,0.0977152118956436,
0.065164916792468));
#5387=CARTESIAN_POINT('Ctrl Pts',(-0.0412904479475092,0.0987224751365548,
0.0653090151899698));
#5388=CARTESIAN_POINT('Ctrl Pts',(-0.0411335425015076,0.0992177720348636,
0.0654121811456859));
#5389=CARTESIAN_POINT('Ctrl Pts',(-0.0405168708018142,0.100636070492068,
0.0657455865368071));
#5390=CARTESIAN_POINT('Ctrl Pts',(-0.039905182689443,0.101492776063005,
0.0659940175331532));
#5391=CARTESIAN_POINT('Ctrl Pts',(-0.0389827504953742,0.102355632371189,
0.0661099450879691));
#5392=CARTESIAN_POINT('Ctrl Pts',(-0.0387729524989471,0.10253278562579,
0.066125));
#5393=CARTESIAN_POINT('Ctrl Pts',(-0.03855,0.1027,0.066125));
#5394=CARTESIAN_POINT('Ctrl Pts',(-0.03855,0.1027,-0.014825));
#5395=CARTESIAN_POINT('Ctrl Pts',(-0.0387729524989471,0.10253278562579,
-0.014825));
#5396=CARTESIAN_POINT('Ctrl Pts',(-0.0389827504953742,0.102355632371189,
-0.0148099450879691));
#5397=CARTESIAN_POINT('Ctrl Pts',(-0.0399051826894431,0.101492776063005,
-0.0146940175331532));
#5398=CARTESIAN_POINT('Ctrl Pts',(-0.0405168708018142,0.100636070492068,
-0.0144455865368071));
#5399=CARTESIAN_POINT('Ctrl Pts',(-0.0411335425015076,0.0992177720348636,
-0.0141121811456859));
#5400=CARTESIAN_POINT('Ctrl Pts',(-0.0412904479475092,0.0987224751365548,
-0.0140090151899698));
#5401=CARTESIAN_POINT('Ctrl Pts',(-0.0414987473161672,0.0977152118956436,
-0.013864916792468));
#5402=CARTESIAN_POINT('Ctrl Pts',(-0.04155,0.0972030713156352,-0.013825));
#5403=CARTESIAN_POINT('Ctrl Pts',(-0.04155,0.0961969286843649,-0.013825));
#5404=CARTESIAN_POINT('Ctrl Pts',(-0.0414987473161672,0.0956847881043564,
-0.013864916792468));
#5405=CARTESIAN_POINT('Ctrl Pts',(-0.0412904479475093,0.0946775248634452,
-0.0140090151899698));
#5406=CARTESIAN_POINT('Ctrl Pts',(-0.0411335425015076,0.0941822279651364,
-0.0141121811456859));
#5407=CARTESIAN_POINT('Ctrl Pts',(-0.0405168708018142,0.0927639295079321,
-0.0144455865368071));
#5408=CARTESIAN_POINT('Ctrl Pts',(-0.0399051826894431,0.0919072239369945,
-0.0146940175331532));
#5409=CARTESIAN_POINT('Ctrl Pts',(-0.0389827504953742,0.0910443676288105,
-0.0148099450879691));
#5410=CARTESIAN_POINT('Ctrl Pts',(-0.0387729524989471,0.0908672143742103,
-0.014825));
#5411=CARTESIAN_POINT('Ctrl Pts',(-0.03855,0.0907,-0.014825));
#5412=CARTESIAN_POINT('Origin',(-0.05605,0.0842,0.003175));
#5413=CARTESIAN_POINT('',(-0.04855,0.0842,0.003175));
#5414=CARTESIAN_POINT('',(-0.06355,0.0842,0.003175));
#5415=CARTESIAN_POINT('Origin',(-0.04355,0.0842,-0.005825));
#5416=CARTESIAN_POINT('',(-0.04355,0.0842,-0.001825));
#5417=CARTESIAN_POINT('',(-0.04355,0.0842,-0.009825));
#5418=CARTESIAN_POINT('Origin',(-0.05605,0.0842,0.048125));
#5419=CARTESIAN_POINT('',(-0.06355,0.0842,0.048125));
#5420=CARTESIAN_POINT('',(-0.04855,0.0842,0.048125));
#5421=CARTESIAN_POINT('Origin',(-0.04355,0.0842,0.057125));
#5422=CARTESIAN_POINT('',(-0.04355,0.0842,0.053125));
#5423=CARTESIAN_POINT('',(-0.04355,0.0842,0.061125));
#5424=CARTESIAN_POINT('Origin',(-0.06355,0.1092,0.008175));
#5425=CARTESIAN_POINT('Origin',(-0.03855,0.0842,-0.009825));
#5426=CARTESIAN_POINT('Origin',(-0.04855,0.0842,-0.001825));
#5427=CARTESIAN_POINT('Origin',(-0.03855,0.1092,0.061125));
#5428=CARTESIAN_POINT('Origin',(-0.04855,0.0842,0.053125));
#5429=CARTESIAN_POINT('Origin',(-0.06355,0.0842,0.043125));
#6301=UNCERTAINTY_MEASURE_WITH_UNIT(LENGTH_MEASURE(1.E-5),#6349,
'DISTANCE_ACCURACY_VALUE',
'Maximum model space distance between geometric entities at asserted c
onnectivities');
#6323=UNCERTAINTY_MEASURE_WITH_UNIT(LENGTH_MEASURE(1.E-5),#6349,
'DISTANCE_ACCURACY_VALUE',
'Maximum model space distance between geometric entities at asserted c
onnectivities');
#6326=(
GEOMETRIC_REPRESENTATION_CONTEXT(3)
GLOBAL_UNCERTAINTY_ASSIGNED_CONTEXT((#6301))
GLOBAL_UNIT_ASSIGNED_CONTEXT((#6349,#6350,#6351))
REPRESENTATION_CONTEXT('','3D')
);
#6348=(
GEOMETRIC_REPRESENTATION_CONTEXT(3)
GLOBAL_UNCERTAINTY_ASSIGNED_CONTEXT((#6323))
GLOBAL_UNIT_ASSIGNED_CONTEXT((#6349,#6350,#6351))
REPRESENTATION_CONTEXT('','3D')
);
#6349=(
LENGTH_UNIT()
NAMED_UNIT(*)
SI_UNIT($,.METRE.)
);
#6350=(
NAMED_UNIT(*)
PLANE_ANGLE_UNIT()
SI_UNIT($,.RADIAN.)
);
#6351=(
NAMED_UNIT(*)
SI_UNIT($,.STERADIAN.)
SOLID_ANGLE_UNIT()
);
#6354=SHAPE_DEFINITION_REPRESENTATION(#6378,#6478);
#6378=PRODUCT_DEFINITION_SHAPE('',$,#6503);
#6478=SHAPE_REPRESENTATION('',(#3562),#6326);
#6500=PRODUCT_DEFINITION_CONTEXT('part definition',#6574,'design');
#6503=PRODUCT_DEFINITION('Back Left Z Mount','Back Left Z Mount',#6527,
#6500);
#6527=PRODUCT_DEFINITION_FORMATION('',$,#6578);
#6574=APPLICATION_CONTEXT('Managed model based 3d engineering');
#6575=PRODUCT_CONTEXT('part definition',#6574,'mechanical');
#6578=PRODUCT('Back Left Z Mount','Back Left Z Mount',
'LEGAL AND USAGE DISCLAIMER: this Data/Model is provided \X2\201C\X0\A
S IS\X2\201D\X0\ for informational and representational only. It is a 
geometric approximation and is NOT engineered, certified, or guarantee
d for dimensional accuracy, exact tolerances, or production-level prec
ision. Vendor disclaims all implied warranties including fitness for a
 particular purpose. DO NOT USE FOR DIRECT PHYSICAL MANUFACTURING, AUT
OMATED PRODUCTION, OR SAFETY-CRITICAL SYSTEMS without independent engi
neering verification and resolution of any design discrepancies.',(#6575));
#6602=PRESENTATION_STYLE_ASSIGNMENT((#6608));
#6608=SURFACE_STYLE_USAGE(.BOTH.,#6614);
#6614=SURFACE_SIDE_STYLE('',(#6620));
#6620=SURFACE_STYLE_FILL_AREA(#6626);
#6626=FILL_AREA_STYLE('Opaque(246,246,243)',(#6632));
#6632=FILL_AREA_STYLE_COLOUR('Opaque(246,246,243)',#6638);
#6638=COLOUR_RGB('Opaque(246,246,243)',0.964705882352941,0.964705882352941,
0.952941176470588);
ENDSEC;
END-ISO-10303-21;
